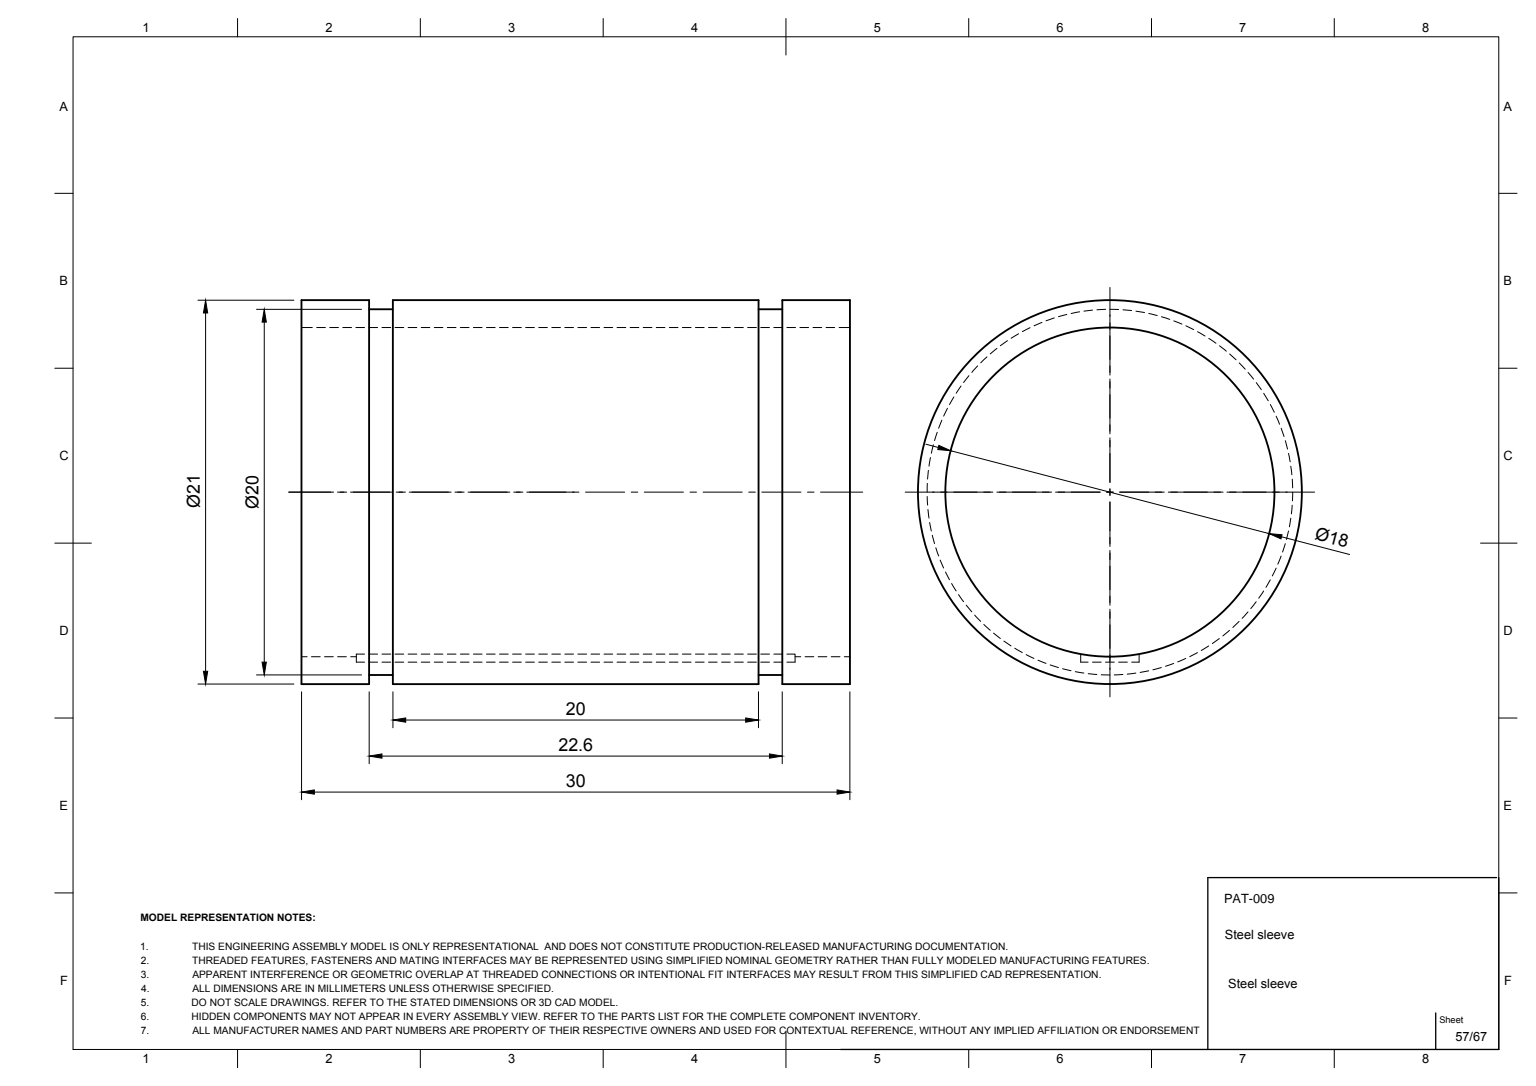
ISO-10303-21;
HEADER;
/* Generated by software containing ST-Developer
 * from STEP Tools, Inc. (www.steptools.com) 
 */

FILE_DESCRIPTION(
/* description */ ('Bell-crank linkage with push rods'),
/* implementation_level */ '2;1');

FILE_NAME(
/* name */ 'Steel sleeve.step',
/* time_stamp */ '2026-10-28T03:25:15-07:00',
/* author */ (''),
/* organization */ (''),
/* preprocessor_version */ 'ST-DEVELOPER v20.2',
/* originating_system */ 'Autodesk Translation Framework v15.17.0.0',
/* authorisation */ '');

FILE_SCHEMA (('AUTOMOTIVE_DESIGN { 1 0 10303 214 3 1 1 }'));
ENDSEC;

DATA;
#10=MECHANICAL_DESIGN_GEOMETRIC_PRESENTATION_REPRESENTATION('',(#663),#16678);
#547=SHAPE_REPRESENTATION_RELATIONSHIP('SRR','None',#16970,#601);
#601=ADVANCED_BREP_SHAPE_REPRESENTATION('',(#723),#16675);
#663=STYLED_ITEM('',(#17305),#723);
#723=MANIFOLD_SOLID_BREP('Body1',#8855);
#954=FACE_BOUND('',#2485,.T.);
#955=FACE_BOUND('',#2488,.T.);
#956=FACE_BOUND('',#2491,.T.);
#957=FACE_BOUND('',#2494,.T.);
#958=FACE_BOUND('',#2497,.T.);
#959=FACE_BOUND('',#2500,.T.);
#960=FACE_BOUND('',#2502,.T.);
#1219=PLANE('',#10468);
#1220=PLANE('',#10470);
#1221=PLANE('',#10471);
#1222=PLANE('',#10473);
#1223=PLANE('',#10474);
#1224=PLANE('',#10475);
#1225=PLANE('',#10480);
#1226=PLANE('',#10484);
#1227=PLANE('',#10488);
#1228=PLANE('',#10492);
#1229=PLANE('',#10496);
#1728=FACE_OUTER_BOUND('',#2479,.T.);
#1729=FACE_OUTER_BOUND('',#2480,.T.);
#1730=FACE_OUTER_BOUND('',#2481,.T.);
#1731=FACE_OUTER_BOUND('',#2482,.T.);
#1732=FACE_OUTER_BOUND('',#2483,.T.);
#1733=FACE_OUTER_BOUND('',#2484,.T.);
#1734=FACE_OUTER_BOUND('',#2486,.T.);
#1735=FACE_OUTER_BOUND('',#2487,.T.);
#1736=FACE_OUTER_BOUND('',#2489,.T.);
#1737=FACE_OUTER_BOUND('',#2490,.T.);
#1738=FACE_OUTER_BOUND('',#2492,.T.);
#1739=FACE_OUTER_BOUND('',#2493,.T.);
#1740=FACE_OUTER_BOUND('',#2495,.T.);
#1741=FACE_OUTER_BOUND('',#2496,.T.);
#1742=FACE_OUTER_BOUND('',#2498,.T.);
#1743=FACE_OUTER_BOUND('',#2499,.T.);
#1744=FACE_OUTER_BOUND('',#2501,.T.);
#2479=EDGE_LOOP('',(#7911,#7912,#7913,#7914));
#2480=EDGE_LOOP('',(#7915,#7916,#7917,#7918));
#2481=EDGE_LOOP('',(#7919,#7920,#7921,#7922));
#2482=EDGE_LOOP('',(#7923,#7924,#7925,#7926));
#2483=EDGE_LOOP('',(#7927,#7928,#7929,#7930));
#2484=EDGE_LOOP('',(#7931));
#2485=EDGE_LOOP('',(#7932));
#2486=EDGE_LOOP('',(#7933,#7934,#7935,#7936));
#2487=EDGE_LOOP('',(#7937));
#2488=EDGE_LOOP('',(#7938));
#2489=EDGE_LOOP('',(#7939,#7940,#7941,#7942));
#2490=EDGE_LOOP('',(#7943));
#2491=EDGE_LOOP('',(#7944));
#2492=EDGE_LOOP('',(#7945,#7946,#7947,#7948));
#2493=EDGE_LOOP('',(#7949));
#2494=EDGE_LOOP('',(#7950));
#2495=EDGE_LOOP('',(#7951,#7952,#7953,#7954));
#2496=EDGE_LOOP('',(#7955));
#2497=EDGE_LOOP('',(#7956));
#2498=EDGE_LOOP('',(#7957,#7958,#7959,#7960));
#2499=EDGE_LOOP('',(#7961));
#2500=EDGE_LOOP('',(#7962));
#2501=EDGE_LOOP('',(#7963,#7964,#7965,#7966));
#2502=EDGE_LOOP('',(#7967,#7968,#7969,#7970));
#3032=LINE('',#16294,#3581);
#3033=LINE('',#16296,#3582);
#3034=LINE('',#16297,#3583);
#3035=LINE('',#16300,#3584);
#3036=LINE('',#16302,#3585);
#3037=LINE('',#16303,#3586);
#3038=LINE('',#16308,#3587);
#3039=LINE('',#16309,#3588);
#3040=LINE('',#16311,#3589);
#3041=LINE('',#16312,#3590);
#3042=LINE('',#16322,#3591);
#3043=LINE('',#16329,#3592);
#3044=LINE('',#16336,#3593);
#3045=LINE('',#16343,#3594);
#3046=LINE('',#16350,#3595);
#3047=LINE('',#16355,#3596);
#3581=VECTOR('',#13162,1.);
#3582=VECTOR('',#13163,1.);
#3583=VECTOR('',#13164,1.);
#3584=VECTOR('',#13167,1.);
#3585=VECTOR('',#13168,1.);
#3586=VECTOR('',#13169,1.);
#3587=VECTOR('',#13174,1.);
#3588=VECTOR('',#13175,1.);
#3589=VECTOR('',#13178,1.);
#3590=VECTOR('',#13179,1.);
#3591=VECTOR('',#13192,1.05);
#3592=VECTOR('',#13201,1.);
#3593=VECTOR('',#13210,1.05);
#3594=VECTOR('',#13219,1.);
#3595=VECTOR('',#13228,1.05);
#3596=VECTOR('',#13235,0.9);
#4091=CIRCLE('',#10469,0.9);
#4092=CIRCLE('',#10472,0.9);
#4093=CIRCLE('',#10476,1.05);
#4094=CIRCLE('',#10477,0.9);
#4095=CIRCLE('',#10479,1.05);
#4096=CIRCLE('',#10481,1.);
#4097=CIRCLE('',#10483,1.);
#4098=CIRCLE('',#10485,1.05);
#4099=CIRCLE('',#10487,1.05);
#4100=CIRCLE('',#10489,1.);
#4101=CIRCLE('',#10491,1.);
#4102=CIRCLE('',#10493,1.05);
#4103=CIRCLE('',#10495,1.05);
#4104=CIRCLE('',#10497,0.9);
#4782=VERTEX_POINT('',#16290);
#4783=VERTEX_POINT('',#16291);
#4784=VERTEX_POINT('',#16293);
#4785=VERTEX_POINT('',#16295);
#4786=VERTEX_POINT('',#16299);
#4787=VERTEX_POINT('',#16301);
#4788=VERTEX_POINT('',#16305);
#4789=VERTEX_POINT('',#16307);
#4790=VERTEX_POINT('',#16315);
#4791=VERTEX_POINT('',#16317);
#4792=VERTEX_POINT('',#16320);
#4793=VERTEX_POINT('',#16324);
#4794=VERTEX_POINT('',#16327);
#4795=VERTEX_POINT('',#16331);
#4796=VERTEX_POINT('',#16334);
#4797=VERTEX_POINT('',#16338);
#4798=VERTEX_POINT('',#16341);
#4799=VERTEX_POINT('',#16345);
#4800=VERTEX_POINT('',#16348);
#4801=VERTEX_POINT('',#16352);
#5833=EDGE_CURVE('',#4782,#4783,#4091,.T.);
#5834=EDGE_CURVE('',#4784,#4782,#3032,.T.);
#5835=EDGE_CURVE('',#4785,#4784,#3033,.T.);
#5836=EDGE_CURVE('',#4783,#4785,#3034,.T.);
#5837=EDGE_CURVE('',#4783,#4786,#3035,.T.);
#5838=EDGE_CURVE('',#4787,#4785,#3036,.T.);
#5839=EDGE_CURVE('',#4787,#4786,#3037,.T.);
#5840=EDGE_CURVE('',#4786,#4788,#4092,.T.);
#5841=EDGE_CURVE('',#4789,#4787,#3038,.T.);
#5842=EDGE_CURVE('',#4788,#4789,#3039,.T.);
#5843=EDGE_CURVE('',#4788,#4782,#3040,.T.);
#5844=EDGE_CURVE('',#4789,#4784,#3041,.T.);
#5845=EDGE_CURVE('',#4790,#4790,#4093,.T.);
#5846=EDGE_CURVE('',#4791,#4791,#4094,.T.);
#5847=EDGE_CURVE('',#4792,#4792,#4095,.T.);
#5848=EDGE_CURVE('',#4792,#4790,#3042,.T.);
#5849=EDGE_CURVE('',#4793,#4793,#4096,.T.);
#5850=EDGE_CURVE('',#4794,#4794,#4097,.T.);
#5851=EDGE_CURVE('',#4794,#4793,#3043,.T.);
#5852=EDGE_CURVE('',#4795,#4795,#4098,.T.);
#5853=EDGE_CURVE('',#4796,#4796,#4099,.T.);
#5854=EDGE_CURVE('',#4796,#4795,#3044,.T.);
#5855=EDGE_CURVE('',#4797,#4797,#4100,.T.);
#5856=EDGE_CURVE('',#4798,#4798,#4101,.T.);
#5857=EDGE_CURVE('',#4798,#4797,#3045,.T.);
#5858=EDGE_CURVE('',#4799,#4799,#4102,.T.);
#5859=EDGE_CURVE('',#4800,#4800,#4103,.T.);
#5860=EDGE_CURVE('',#4800,#4799,#3046,.T.);
#5861=EDGE_CURVE('',#4801,#4801,#4104,.T.);
#5862=EDGE_CURVE('',#4801,#4791,#3047,.T.);
#7911=ORIENTED_EDGE('',*,*,#5833,.F.);
#7912=ORIENTED_EDGE('',*,*,#5834,.F.);
#7913=ORIENTED_EDGE('',*,*,#5835,.F.);
#7914=ORIENTED_EDGE('',*,*,#5836,.F.);
#7915=ORIENTED_EDGE('',*,*,#5837,.F.);
#7916=ORIENTED_EDGE('',*,*,#5836,.T.);
#7917=ORIENTED_EDGE('',*,*,#5838,.F.);
#7918=ORIENTED_EDGE('',*,*,#5839,.T.);
#7919=ORIENTED_EDGE('',*,*,#5840,.F.);
#7920=ORIENTED_EDGE('',*,*,#5839,.F.);
#7921=ORIENTED_EDGE('',*,*,#5841,.F.);
#7922=ORIENTED_EDGE('',*,*,#5842,.F.);
#7923=ORIENTED_EDGE('',*,*,#5843,.F.);
#7924=ORIENTED_EDGE('',*,*,#5842,.T.);
#7925=ORIENTED_EDGE('',*,*,#5844,.T.);
#7926=ORIENTED_EDGE('',*,*,#5834,.T.);
#7927=ORIENTED_EDGE('',*,*,#5844,.F.);
#7928=ORIENTED_EDGE('',*,*,#5841,.T.);
#7929=ORIENTED_EDGE('',*,*,#5838,.T.);
#7930=ORIENTED_EDGE('',*,*,#5835,.T.);
#7931=ORIENTED_EDGE('',*,*,#5845,.F.);
#7932=ORIENTED_EDGE('',*,*,#5846,.T.);
#7933=ORIENTED_EDGE('',*,*,#5847,.F.);
#7934=ORIENTED_EDGE('',*,*,#5848,.T.);
#7935=ORIENTED_EDGE('',*,*,#5845,.T.);
#7936=ORIENTED_EDGE('',*,*,#5848,.F.);
#7937=ORIENTED_EDGE('',*,*,#5847,.T.);
#7938=ORIENTED_EDGE('',*,*,#5849,.F.);
#7939=ORIENTED_EDGE('',*,*,#5850,.F.);
#7940=ORIENTED_EDGE('',*,*,#5851,.T.);
#7941=ORIENTED_EDGE('',*,*,#5849,.T.);
#7942=ORIENTED_EDGE('',*,*,#5851,.F.);
#7943=ORIENTED_EDGE('',*,*,#5852,.F.);
#7944=ORIENTED_EDGE('',*,*,#5850,.T.);
#7945=ORIENTED_EDGE('',*,*,#5853,.F.);
#7946=ORIENTED_EDGE('',*,*,#5854,.T.);
#7947=ORIENTED_EDGE('',*,*,#5852,.T.);
#7948=ORIENTED_EDGE('',*,*,#5854,.F.);
#7949=ORIENTED_EDGE('',*,*,#5853,.T.);
#7950=ORIENTED_EDGE('',*,*,#5855,.F.);
#7951=ORIENTED_EDGE('',*,*,#5856,.F.);
#7952=ORIENTED_EDGE('',*,*,#5857,.T.);
#7953=ORIENTED_EDGE('',*,*,#5855,.T.);
#7954=ORIENTED_EDGE('',*,*,#5857,.F.);
#7955=ORIENTED_EDGE('',*,*,#5858,.F.);
#7956=ORIENTED_EDGE('',*,*,#5856,.T.);
#7957=ORIENTED_EDGE('',*,*,#5859,.F.);
#7958=ORIENTED_EDGE('',*,*,#5860,.T.);
#7959=ORIENTED_EDGE('',*,*,#5858,.T.);
#7960=ORIENTED_EDGE('',*,*,#5860,.F.);
#7961=ORIENTED_EDGE('',*,*,#5859,.T.);
#7962=ORIENTED_EDGE('',*,*,#5861,.F.);
#7963=ORIENTED_EDGE('',*,*,#5861,.T.);
#7964=ORIENTED_EDGE('',*,*,#5862,.T.);
#7965=ORIENTED_EDGE('',*,*,#5846,.F.);
#7966=ORIENTED_EDGE('',*,*,#5862,.F.);
#7967=ORIENTED_EDGE('',*,*,#5840,.T.);
#7968=ORIENTED_EDGE('',*,*,#5843,.T.);
#7969=ORIENTED_EDGE('',*,*,#5833,.T.);
#7970=ORIENTED_EDGE('',*,*,#5837,.T.);
#8262=CYLINDRICAL_SURFACE('',#10478,1.05);
#8263=CYLINDRICAL_SURFACE('',#10482,1.);
#8264=CYLINDRICAL_SURFACE('',#10486,1.05);
#8265=CYLINDRICAL_SURFACE('',#10490,1.);
#8266=CYLINDRICAL_SURFACE('',#10494,1.05);
#8267=CYLINDRICAL_SURFACE('',#10498,0.9);
#8753=ADVANCED_FACE('',(#1728),#1219,.F.);
#8754=ADVANCED_FACE('',(#1729),#1220,.F.);
#8755=ADVANCED_FACE('',(#1730),#1221,.F.);
#8756=ADVANCED_FACE('',(#1731),#1222,.F.);
#8757=ADVANCED_FACE('',(#1732),#1223,.F.);
#8758=ADVANCED_FACE('',(#1733,#954),#1224,.T.);
#8759=ADVANCED_FACE('',(#1734),#8262,.T.);
#8760=ADVANCED_FACE('',(#1735,#955),#1225,.T.);
#8761=ADVANCED_FACE('',(#1736),#8263,.T.);
#8762=ADVANCED_FACE('',(#1737,#956),#1226,.T.);
#8763=ADVANCED_FACE('',(#1738),#8264,.T.);
#8764=ADVANCED_FACE('',(#1739,#957),#1227,.T.);
#8765=ADVANCED_FACE('',(#1740),#8265,.T.);
#8766=ADVANCED_FACE('',(#1741,#958),#1228,.T.);
#8767=ADVANCED_FACE('',(#1742),#8266,.T.);
#8768=ADVANCED_FACE('',(#1743,#959),#1229,.T.);
#8769=ADVANCED_FACE('',(#1744,#960),#8267,.F.);
#8855=CLOSED_SHELL('',(#8753,#8754,#8755,#8756,#8757,#8758,#8759,#8760,
#8761,#8762,#8763,#8764,#8765,#8766,#8767,#8768,#8769));
#10467=AXIS2_PLACEMENT_3D('',#16288,#13156,#13157);
#10468=AXIS2_PLACEMENT_3D('',#16289,#13158,#13159);
#10469=AXIS2_PLACEMENT_3D('',#16292,#13160,#13161);
#10470=AXIS2_PLACEMENT_3D('',#16298,#13165,#13166);
#10471=AXIS2_PLACEMENT_3D('',#16304,#13170,#13171);
#10472=AXIS2_PLACEMENT_3D('',#16306,#13172,#13173);
#10473=AXIS2_PLACEMENT_3D('',#16310,#13176,#13177);
#10474=AXIS2_PLACEMENT_3D('',#16313,#13180,#13181);
#10475=AXIS2_PLACEMENT_3D('',#16314,#13182,#13183);
#10476=AXIS2_PLACEMENT_3D('',#16316,#13184,#13185);
#10477=AXIS2_PLACEMENT_3D('',#16318,#13186,#13187);
#10478=AXIS2_PLACEMENT_3D('',#16319,#13188,#13189);
#10479=AXIS2_PLACEMENT_3D('',#16321,#13190,#13191);
#10480=AXIS2_PLACEMENT_3D('',#16323,#13193,#13194);
#10481=AXIS2_PLACEMENT_3D('',#16325,#13195,#13196);
#10482=AXIS2_PLACEMENT_3D('',#16326,#13197,#13198);
#10483=AXIS2_PLACEMENT_3D('',#16328,#13199,#13200);
#10484=AXIS2_PLACEMENT_3D('',#16330,#13202,#13203);
#10485=AXIS2_PLACEMENT_3D('',#16332,#13204,#13205);
#10486=AXIS2_PLACEMENT_3D('',#16333,#13206,#13207);
#10487=AXIS2_PLACEMENT_3D('',#16335,#13208,#13209);
#10488=AXIS2_PLACEMENT_3D('',#16337,#13211,#13212);
#10489=AXIS2_PLACEMENT_3D('',#16339,#13213,#13214);
#10490=AXIS2_PLACEMENT_3D('',#16340,#13215,#13216);
#10491=AXIS2_PLACEMENT_3D('',#16342,#13217,#13218);
#10492=AXIS2_PLACEMENT_3D('',#16344,#13220,#13221);
#10493=AXIS2_PLACEMENT_3D('',#16346,#13222,#13223);
#10494=AXIS2_PLACEMENT_3D('',#16347,#13224,#13225);
#10495=AXIS2_PLACEMENT_3D('',#16349,#13226,#13227);
#10496=AXIS2_PLACEMENT_3D('',#16351,#13229,#13230);
#10497=AXIS2_PLACEMENT_3D('',#16353,#13231,#13232);
#10498=AXIS2_PLACEMENT_3D('',#16354,#13233,#13234);
#13156=DIRECTION('axis',(0.,0.,1.));
#13157=DIRECTION('refdir',(1.,0.,0.));
#13158=DIRECTION('center_axis',(0.,1.,0.));
#13159=DIRECTION('ref_axis',(0.,0.,1.));
#13160=DIRECTION('center_axis',(0.,-1.,0.));
#13161=DIRECTION('ref_axis',(1.,0.,0.));
#13162=DIRECTION('',(-1.,0.,0.));
#13163=DIRECTION('',(0.,0.,-1.));
#13164=DIRECTION('',(1.,0.,0.));
#13165=DIRECTION('center_axis',(0.,0.,1.));
#13166=DIRECTION('ref_axis',(1.,0.,0.));
#13167=DIRECTION('',(0.,-1.,0.));
#13168=DIRECTION('',(0.,1.,0.));
#13169=DIRECTION('',(-1.,0.,0.));
#13170=DIRECTION('center_axis',(0.,-1.,0.));
#13171=DIRECTION('ref_axis',(0.,0.,-1.));
#13172=DIRECTION('center_axis',(0.,1.,0.));
#13173=DIRECTION('ref_axis',(1.,0.,0.));
#13174=DIRECTION('',(0.,0.,1.));
#13175=DIRECTION('',(1.,0.,0.));
#13176=DIRECTION('center_axis',(0.,0.,-1.));
#13177=DIRECTION('ref_axis',(-1.,0.,0.));
#13178=DIRECTION('',(0.,1.,0.));
#13179=DIRECTION('',(0.,1.,0.));
#13180=DIRECTION('center_axis',(1.,0.,0.));
#13181=DIRECTION('ref_axis',(0.,0.,-1.));
#13182=DIRECTION('center_axis',(0.,1.,0.));
#13183=DIRECTION('ref_axis',(0.,0.,1.));
#13184=DIRECTION('center_axis',(0.,-1.,0.));
#13185=DIRECTION('ref_axis',(1.,0.,0.));
#13186=DIRECTION('center_axis',(0.,-1.,0.));
#13187=DIRECTION('ref_axis',(1.,0.,0.));
#13188=DIRECTION('center_axis',(0.,-1.,0.));
#13189=DIRECTION('ref_axis',(1.,0.,0.));
#13190=DIRECTION('center_axis',(0.,-1.,0.));
#13191=DIRECTION('ref_axis',(1.,0.,0.));
#13192=DIRECTION('',(0.,1.,0.));
#13193=DIRECTION('center_axis',(0.,-1.,0.));
#13194=DIRECTION('ref_axis',(0.,0.,-1.));
#13195=DIRECTION('center_axis',(0.,-1.,0.));
#13196=DIRECTION('ref_axis',(1.,0.,0.));
#13197=DIRECTION('center_axis',(0.,-1.,0.));
#13198=DIRECTION('ref_axis',(1.,0.,0.));
#13199=DIRECTION('center_axis',(0.,-1.,0.));
#13200=DIRECTION('ref_axis',(1.,0.,0.));
#13201=DIRECTION('',(0.,1.,0.));
#13202=DIRECTION('center_axis',(0.,1.,0.));
#13203=DIRECTION('ref_axis',(0.,0.,1.));
#13204=DIRECTION('center_axis',(0.,-1.,0.));
#13205=DIRECTION('ref_axis',(1.,0.,0.));
#13206=DIRECTION('center_axis',(0.,-1.,0.));
#13207=DIRECTION('ref_axis',(1.,0.,0.));
#13208=DIRECTION('center_axis',(0.,-1.,0.));
#13209=DIRECTION('ref_axis',(1.,0.,0.));
#13210=DIRECTION('',(0.,1.,0.));
#13211=DIRECTION('center_axis',(0.,-1.,0.));
#13212=DIRECTION('ref_axis',(0.,0.,-1.));
#13213=DIRECTION('center_axis',(0.,-1.,0.));
#13214=DIRECTION('ref_axis',(1.,0.,0.));
#13215=DIRECTION('center_axis',(0.,-1.,0.));
#13216=DIRECTION('ref_axis',(1.,0.,0.));
#13217=DIRECTION('center_axis',(0.,-1.,0.));
#13218=DIRECTION('ref_axis',(1.,0.,0.));
#13219=DIRECTION('',(0.,1.,0.));
#13220=DIRECTION('center_axis',(0.,1.,0.));
#13221=DIRECTION('ref_axis',(0.,0.,1.));
#13222=DIRECTION('center_axis',(0.,-1.,0.));
#13223=DIRECTION('ref_axis',(1.,0.,0.));
#13224=DIRECTION('center_axis',(0.,-1.,0.));
#13225=DIRECTION('ref_axis',(1.,0.,0.));
#13226=DIRECTION('center_axis',(0.,-1.,0.));
#13227=DIRECTION('ref_axis',(1.,0.,0.));
#13228=DIRECTION('',(0.,1.,0.));
#13229=DIRECTION('center_axis',(0.,-1.,0.));
#13230=DIRECTION('ref_axis',(0.,0.,-1.));
#13231=DIRECTION('center_axis',(0.,-1.,0.));
#13232=DIRECTION('ref_axis',(1.,0.,0.));
#13233=DIRECTION('center_axis',(0.,-1.,0.));
#13234=DIRECTION('ref_axis',(1.,0.,0.));
#13235=DIRECTION('',(0.,1.,0.));
#16288=CARTESIAN_POINT('',(0.,0.,0.));
#16289=CARTESIAN_POINT('Origin',(0.75,1.2,0.));
#16290=CARTESIAN_POINT('',(0.885663593019381,1.2,-0.16));
#16291=CARTESIAN_POINT('',(0.885663593019381,1.2,0.16));
#16292=CARTESIAN_POINT('Origin',(0.,1.2,0.));
#16293=CARTESIAN_POINT('',(0.93,1.2,-0.16));
#16294=CARTESIAN_POINT('',(0.93,1.2,-0.16));
#16295=CARTESIAN_POINT('',(0.93,1.2,0.16));
#16296=CARTESIAN_POINT('',(0.93,1.2,0.16));
#16297=CARTESIAN_POINT('',(0.57,1.2,0.16));
#16298=CARTESIAN_POINT('Origin',(0.57,0.,0.16));
#16299=CARTESIAN_POINT('',(0.885663593019381,-1.2,0.16));
#16300=CARTESIAN_POINT('',(0.885663593019381,0.,0.16));
#16301=CARTESIAN_POINT('',(0.93,-1.2,0.16));
#16302=CARTESIAN_POINT('',(0.93,0.,0.16));
#16303=CARTESIAN_POINT('',(0.57,-1.2,0.16));
#16304=CARTESIAN_POINT('Origin',(0.75,-1.2,0.));
#16305=CARTESIAN_POINT('',(0.885663593019381,-1.2,-0.16));
#16306=CARTESIAN_POINT('Origin',(0.,-1.2,0.));
#16307=CARTESIAN_POINT('',(0.93,-1.2,-0.16));
#16308=CARTESIAN_POINT('',(0.93,-1.2,0.16));
#16309=CARTESIAN_POINT('',(0.93,-1.2,-0.16));
#16310=CARTESIAN_POINT('Origin',(0.93,0.,-0.16));
#16311=CARTESIAN_POINT('',(0.885663593019381,0.,-0.16));
#16312=CARTESIAN_POINT('',(0.93,0.,-0.16));
#16313=CARTESIAN_POINT('Origin',(0.93,0.,0.16));
#16314=CARTESIAN_POINT('Origin',(1.05,1.5,0.));
#16315=CARTESIAN_POINT('',(-1.05,1.5,-1.28587913910472E-16));
#16316=CARTESIAN_POINT('Origin',(0.,1.5,0.));
#16317=CARTESIAN_POINT('',(-0.9,1.5,-1.10218211923262E-16));
#16318=CARTESIAN_POINT('Origin',(0.,1.5,0.));
#16319=CARTESIAN_POINT('Origin',(0.,1.315,0.));
#16320=CARTESIAN_POINT('',(-1.05,1.13,-1.28587913910472E-16));
#16321=CARTESIAN_POINT('Origin',(0.,1.13,0.));
#16322=CARTESIAN_POINT('',(-1.05,1.315,-1.28587913910472E-16));
#16323=CARTESIAN_POINT('Origin',(1.,1.13,0.));
#16324=CARTESIAN_POINT('',(-1.,1.13,-1.22464679914735E-16));
#16325=CARTESIAN_POINT('Origin',(0.,1.13,0.));
#16326=CARTESIAN_POINT('Origin',(0.,1.065,0.));
#16327=CARTESIAN_POINT('',(-1.,1.,-1.22464679914735E-16));
#16328=CARTESIAN_POINT('Origin',(0.,1.,0.));
#16329=CARTESIAN_POINT('',(-1.,1.065,-1.22464679914735E-16));
#16330=CARTESIAN_POINT('Origin',(1.05,1.,0.));
#16331=CARTESIAN_POINT('',(-1.05,1.,-1.28587913910472E-16));
#16332=CARTESIAN_POINT('Origin',(0.,1.,0.));
#16333=CARTESIAN_POINT('Origin',(0.,0.,0.));
#16334=CARTESIAN_POINT('',(-1.05,-1.,-1.28587913910472E-16));
#16335=CARTESIAN_POINT('Origin',(0.,-1.,0.));
#16336=CARTESIAN_POINT('',(-1.05,0.,-1.28587913910472E-16));
#16337=CARTESIAN_POINT('Origin',(1.,-1.,0.));
#16338=CARTESIAN_POINT('',(-1.,-1.,-1.22464679914735E-16));
#16339=CARTESIAN_POINT('Origin',(0.,-1.,0.));
#16340=CARTESIAN_POINT('Origin',(0.,-1.065,0.));
#16341=CARTESIAN_POINT('',(-1.,-1.13,-1.22464679914735E-16));
#16342=CARTESIAN_POINT('Origin',(0.,-1.13,0.));
#16343=CARTESIAN_POINT('',(-1.,-1.065,-1.22464679914735E-16));
#16344=CARTESIAN_POINT('Origin',(1.05,-1.13,0.));
#16345=CARTESIAN_POINT('',(-1.05,-1.13,-1.28587913910472E-16));
#16346=CARTESIAN_POINT('Origin',(0.,-1.13,0.));
#16347=CARTESIAN_POINT('Origin',(0.,-1.315,0.));
#16348=CARTESIAN_POINT('',(-1.05,-1.5,-1.28587913910472E-16));
#16349=CARTESIAN_POINT('Origin',(0.,-1.5,0.));
#16350=CARTESIAN_POINT('',(-1.05,-1.315,-1.28587913910472E-16));
#16351=CARTESIAN_POINT('Origin',(0.9,-1.5,0.));
#16352=CARTESIAN_POINT('',(-0.9,-1.5,-1.10218211923262E-16));
#16353=CARTESIAN_POINT('Origin',(0.,-1.5,0.));
#16354=CARTESIAN_POINT('Origin',(0.,0.,0.));
#16355=CARTESIAN_POINT('',(-0.9,0.,-1.10218211923262E-16));
#16611=UNCERTAINTY_MEASURE_WITH_UNIT(LENGTH_MEASURE(0.001),#16679,
'DISTANCE_ACCURACY_VALUE',
'Maximum model space distance between geometric entities at asserted c
onnectivities');
#16614=UNCERTAINTY_MEASURE_WITH_UNIT(LENGTH_MEASURE(0.001),#16679,
'DISTANCE_ACCURACY_VALUE',
'Maximum model space distance between geometric entities at asserted c
onnectivities');
#16675=(
GEOMETRIC_REPRESENTATION_CONTEXT(3)
GLOBAL_UNCERTAINTY_ASSIGNED_CONTEXT((#16611))
GLOBAL_UNIT_ASSIGNED_CONTEXT((#16679,#16681,#16682))
REPRESENTATION_CONTEXT('','3D')
);
#16678=(
GEOMETRIC_REPRESENTATION_CONTEXT(3)
GLOBAL_UNCERTAINTY_ASSIGNED_CONTEXT((#16614))
GLOBAL_UNIT_ASSIGNED_CONTEXT((#16679,#16681,#16682))
REPRESENTATION_CONTEXT('','3D')
);
#16679=(
LENGTH_UNIT()
NAMED_UNIT(*)
SI_UNIT(.CENTI.,.METRE.)
);
#16681=(
NAMED_UNIT(*)
PLANE_ANGLE_UNIT()
SI_UNIT($,.RADIAN.)
);
#16682=(
NAMED_UNIT(*)
SI_UNIT($,.STERADIAN.)
SOLID_ANGLE_UNIT()
);
#16743=SHAPE_DEFINITION_REPRESENTATION(#16817,#16970);
#16817=PRODUCT_DEFINITION_SHAPE('',$,#17034);
#16970=SHAPE_REPRESENTATION('',(#10467),#16675);
#16973=PRODUCT_DEFINITION_CONTEXT('part definition',#17164,'design');
#17034=PRODUCT_DEFINITION('Steel sleeve','Steel sleeve',#17097,#16973);
#17097=PRODUCT_DEFINITION_FORMATION('',$,#17226);
#17164=APPLICATION_CONTEXT(
'Core Data for Automotive Mechanical Design Process');
#17165=PRODUCT_CONTEXT('part definition',#17164,'mechanical');
#17226=PRODUCT('Steel sleeve','Steel sleeve','Steel sleeve',(#17165));
#17299=COLOUR_RGB('Off White',0.89,0.88,0.83);
#17300=FILL_AREA_STYLE_COLOUR('',#17299);
#17301=FILL_AREA_STYLE('',(#17300));
#17302=SURFACE_STYLE_FILL_AREA(#17301);
#17303=SURFACE_SIDE_STYLE('',(#17302));
#17304=SURFACE_STYLE_USAGE(.BOTH.,#17303);
#17305=PRESENTATION_STYLE_ASSIGNMENT((#17304));
ENDSEC;
END-ISO-10303-21;
